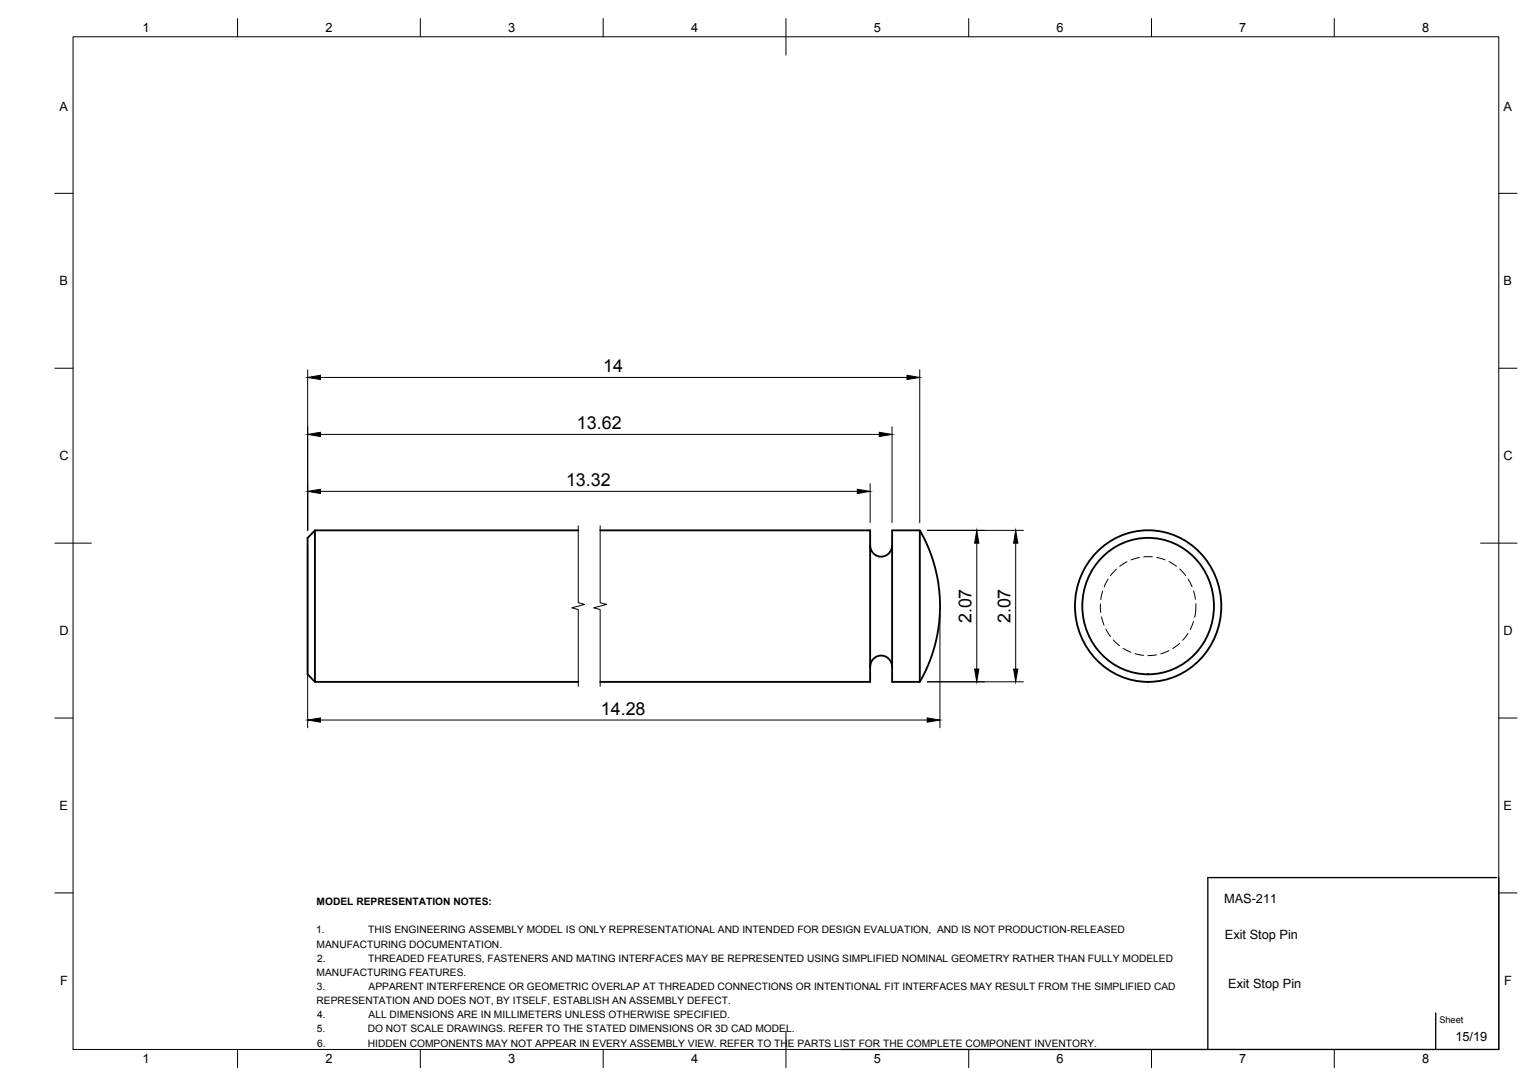
ISO-10303-21;
HEADER;
FILE_DESCRIPTION(
 (''),
 '2;1');
FILE_NAME ( 'Exit Stop Pin.step', '2026-10-05T20:07:59+06:00', ( '' ), ( '' ), 'STEP AP214', 'Unspecified', '' );
FILE_SCHEMA (('AUTOMOTIVE_DESIGN { 1 0 10303 214 3 1 1 }'));
ENDSEC;
DATA;
#10=MECHANICAL_DESIGN_GEOMETRIC_PRESENTATION_REPRESENTATION('',(#333),#196741);
#26=(
BOUNDED_CURVE()
B_SPLINE_CURVE(2,(#154684,#154685,#154686,#154687,#154688,#154689,#154690,
#154691,#154692),.UNSPECIFIED.,.F.,.F.)
B_SPLINE_CURVE_WITH_KNOTS((3,2,2,2,3),(1.42918797785348,1.62618617063892,
1.86180561965816,2.09742506867739,2.29442326146283),.UNSPECIFIED.)
CURVE()
GEOMETRIC_REPRESENTATION_ITEM()
RATIONAL_B_SPLINE_CURVE((1.,1.,1.,0.707106781186548,1.,0.707106781186548,
1.,1.,1.))
REPRESENTATION_ITEM('')
) ;
#56=(
BOUNDED_SURFACE()
B_SPLINE_SURFACE(2,2,((#154549,#154550,#154551,#154552,#154553,#154554,
#154555,#154556,#154557),(#154558,#154559,#154560,#154561,#154562,#154563,
#154564,#154565,#154566),(#154567,#154568,#154569,#154570,#154571,#154572,
#154573,#154574,#154575)),.UNSPECIFIED.,.F.,.T.,.F.)
B_SPLINE_SURFACE_WITH_KNOTS((3,3),(3,2,2,2,3),(0.,1.05013832301181),(0.,
1.5707963267949,3.1415926535898,4.71238898038469,6.28318530717959),
 .UNSPECIFIED.)
GEOMETRIC_REPRESENTATION_ITEM()
RATIONAL_B_SPLINE_SURFACE(((1.,0.707106781186548,1.,0.707106781186548,1.,
0.707106781186548,1.,0.707106781186548,1.),(0.963886720506905,0.681570836366095,
0.963886720506905,0.681570836366095,0.963886720506905,0.681570836366095,
0.963886720506905,0.681570836366095,0.963886720506905),(1.,0.707106781186548,
1.,0.707106781186548,1.,0.707106781186548,1.,0.707106781186548,1.)))
REPRESENTATION_ITEM('')
SURFACE()
) ;
#57=(
BOUNDED_SURFACE()
B_SPLINE_SURFACE(2,1,((#154580,#154581),(#154582,#154583),(#154584,#154585),
(#154586,#154587),(#154588,#154589),(#154590,#154591),(#154592,#154593),
(#154594,#154595),(#154596,#154597)),.UNSPECIFIED.,.T.,.F.,.F.)
B_SPLINE_SURFACE_WITH_KNOTS((3,2,2,2,3),(2,2),(0.,1.5707963267949,3.1415926535898,
4.71238898038469,6.28318530717959),(0.,0.0454859585810007),
 .UNSPECIFIED.)
GEOMETRIC_REPRESENTATION_ITEM()
RATIONAL_B_SPLINE_SURFACE(((1.,1.),(0.707106781186548,0.707106781186548),
(1.,1.),(0.707106781186548,0.707106781186548),(1.,1.),(0.707106781186548,
0.707106781186548),(1.,1.),(0.707106781186548,0.707106781186548),(1.,1.)))
REPRESENTATION_ITEM('')
SURFACE()
) ;
#58=(
BOUNDED_SURFACE()
B_SPLINE_SURFACE(2,2,((#154601,#154602,#154603,#154604,#154605,#154606,
#154607,#154608,#154609),(#154610,#154611,#154612,#154613,#154614,#154615,
#154616,#154617,#154618),(#154619,#154620,#154621,#154622,#154623,#154624,
#154625,#154626,#154627),(#154628,#154629,#154630,#154631,#154632,#154633,
#154634,#154635,#154636),(#154637,#154638,#154639,#154640,#154641,#154642,
#154643,#154644,#154645),(#154646,#154647,#154648,#154649,#154650,#154651,
#154652,#154653,#154654),(#154655,#154656,#154657,#154658,#154659,#154660,
#154661,#154662,#154663),(#154664,#154665,#154666,#154667,#154668,#154669,
#154670,#154671,#154672),(#154673,#154674,#154675,#154676,#154677,#154678,
#154679,#154680,#154681)),.UNSPECIFIED.,.F.,.T.,.F.)
B_SPLINE_SURFACE_WITH_KNOTS((3,2,2,2,3),(3,2,2,2,3),(1.42918797785348,1.62618617063892,
1.86180561965816,2.09742506867739,2.29442326146283),(0.,1.5707963267949,
3.1415926535898,4.71238898038469,6.28318530717959),.UNSPECIFIED.)
GEOMETRIC_REPRESENTATION_ITEM()
RATIONAL_B_SPLINE_SURFACE(((1.,0.707106781186548,1.,0.707106781186548,1.,
0.707106781186548,1.,0.707106781186548,1.),(1.,0.707106781186548,1.,0.707106781186548,
1.,0.707106781186548,1.,0.707106781186548,1.),(1.,0.707106781186548,1.,
0.707106781186548,1.,0.707106781186548,1.,0.707106781186548,1.),(0.707106781186548,
0.5,0.707106781186548,0.5,0.707106781186548,0.5,0.707106781186548,0.5,0.707106781186548),
(1.,0.707106781186548,1.,0.707106781186548,1.,0.707106781186548,1.,0.707106781186548,
1.),(0.707106781186548,0.5,0.707106781186548,0.5,0.707106781186548,0.5,
0.707106781186548,0.5,0.707106781186548),(1.,0.707106781186548,1.,0.707106781186548,
1.,0.707106781186548,1.,0.707106781186548,1.),(1.,0.707106781186548,1.,
0.707106781186548,1.,0.707106781186548,1.,0.707106781186548,1.),(1.,0.707106781186548,
1.,0.707106781186548,1.,0.707106781186548,1.,0.707106781186548,1.)))
REPRESENTATION_ITEM('')
SURFACE()
) ;
#59=(
BOUNDED_SURFACE()
B_SPLINE_SURFACE(2,1,((#154693,#154694),(#154695,#154696),(#154697,#154698),
(#154699,#154700),(#154701,#154702),(#154703,#154704),(#154705,#154706),
(#154707,#154708),(#154709,#154710)),.UNSPECIFIED.,.T.,.F.,.F.)
B_SPLINE_SURFACE_WITH_KNOTS((3,2,2,2,3),(2,2),(0.,1.5707963267949,3.1415926535898,
4.71238898038469,6.28318530717959),(0.,1.586514041419),.UNSPECIFIED.)
GEOMETRIC_REPRESENTATION_ITEM()
RATIONAL_B_SPLINE_SURFACE(((1.,1.),(0.707106781186548,0.707106781186548),
(1.,1.),(0.707106781186548,0.707106781186548),(1.,1.),(0.707106781186548,
0.707106781186548),(1.,1.),(0.707106781186548,0.707106781186548),(1.,1.)))
REPRESENTATION_ITEM('')
SURFACE()
) ;
#60=(
BOUNDED_SURFACE()
B_SPLINE_SURFACE(1,2,((#154714,#154715,#154716,#154717,#154718,#154719,
#154720,#154721,#154722),(#154723,#154724,#154725,#154726,#154727,#154728,
#154729,#154730,#154731)),.UNSPECIFIED.,.F.,.T.,.F.)
B_SPLINE_SURFACE_WITH_KNOTS((2,2),(3,2,2,2,3),(15.5153736066212,15.6567949628585),
(0.,1.5707963267949,3.1415926535898,4.71238898038469,6.28318530717959),
 .UNSPECIFIED.)
GEOMETRIC_REPRESENTATION_ITEM()
RATIONAL_B_SPLINE_SURFACE(((1.,0.707106781186548,1.,0.707106781186548,1.,
0.707106781186548,1.,0.707106781186548,1.),(1.,0.707106781186548,1.,0.707106781186548,
1.,0.707106781186548,1.,0.707106781186548,1.)))
REPRESENTATION_ITEM('')
SURFACE()
) ;
#170=ELLIPSE('',#9016,0.932157550311782,0.900000000000012) ;
#171=ELLIPSE('',#9017,1.03573061145752,1.) ;
#172=ELLIPSE('',#9019,1.03573061145752,1.) ;
#173=ELLIPSE('',#9020,1.03573061145752,1.) ;
#174=ELLIPSE('',#9021,1.03573061145752,1.) ;
#333=STYLED_ITEM('',(#196765),#352) ;
#352=MANIFOLD_SOLID_BREP('Exit Stop Pin',#8729) ;
#405=PLANE('',#9015) ;
#710=CIRCLE('',#9018,1.94783572104112) ;
#1060=FACE_OUTER_BOUND('',#1569,.T.) ;
#1061=FACE_OUTER_BOUND('',#1570,.T.) ;
#1062=FACE_OUTER_BOUND('',#1571,.T.) ;
#1063=FACE_OUTER_BOUND('',#1572,.T.) ;
#1064=FACE_OUTER_BOUND('',#1573,.T.) ;
#1065=FACE_OUTER_BOUND('',#1574,.T.) ;
#1569=EDGE_LOOP('',(#6574,#6575,#6576)) ;
#1570=EDGE_LOOP('',(#6577,#6578,#6579)) ;
#1571=EDGE_LOOP('',(#6580,#6581,#6582,#6583)) ;
#1572=EDGE_LOOP('',(#6584,#6585,#6586,#6587)) ;
#1573=EDGE_LOOP('',(#6588,#6589,#6590,#6591)) ;
#1574=EDGE_LOOP('',(#6592,#6593,#6594,#6595)) ;
#2048=LINE('',#154547,#2751) ;
#2049=LINE('',#154600,#2752) ;
#2050=LINE('',#154713,#2753) ;
#2051=LINE('',#154732,#2754) ;
#2751=VECTOR('',#10180,10.) ;
#2752=VECTOR('',#10189,10.) ;
#2753=VECTOR('',#10194,10.) ;
#2754=VECTOR('',#10195,10.) ;
#3777=VERTEX_POINT('',#154545) ;
#3778=VERTEX_POINT('',#154546) ;
#3779=VERTEX_POINT('',#154576) ;
#3780=VERTEX_POINT('',#154578) ;
#3781=VERTEX_POINT('',#154598) ;
#3782=VERTEX_POINT('',#154682) ;
#3783=VERTEX_POINT('',#154711) ;
#4795=EDGE_CURVE('',#3777,#3778,#2048,.T.) ;
#4796=EDGE_CURVE('',#3777,#3777,#170,.T.) ;
#4797=EDGE_CURVE('',#3779,#3779,#171,.T.) ;
#4798=EDGE_CURVE('',#3780,#3779,#710,.T.) ;
#4799=EDGE_CURVE('',#3781,#3781,#172,.T.) ;
#4800=EDGE_CURVE('',#3779,#3781,#2049,.T.) ;
#4801=EDGE_CURVE('',#3782,#3782,#173,.T.) ;
#4802=EDGE_CURVE('',#3781,#3782,#26,.T.) ;
#4803=EDGE_CURVE('',#3783,#3783,#174,.T.) ;
#4804=EDGE_CURVE('',#3782,#3783,#2050,.T.) ;
#4805=EDGE_CURVE('',#3783,#3777,#2051,.T.) ;
#6574=ORIENTED_EDGE('',*,*,#4795,.T.) ;
#6575=ORIENTED_EDGE('',*,*,#4795,.F.) ;
#6576=ORIENTED_EDGE('',*,*,#4796,.F.) ;
#6577=ORIENTED_EDGE('',*,*,#4797,.T.) ;
#6578=ORIENTED_EDGE('',*,*,#4798,.F.) ;
#6579=ORIENTED_EDGE('',*,*,#4798,.T.) ;
#6580=ORIENTED_EDGE('',*,*,#4799,.T.) ;
#6581=ORIENTED_EDGE('',*,*,#4800,.F.) ;
#6582=ORIENTED_EDGE('',*,*,#4797,.F.) ;
#6583=ORIENTED_EDGE('',*,*,#4800,.T.) ;
#6584=ORIENTED_EDGE('',*,*,#4801,.T.) ;
#6585=ORIENTED_EDGE('',*,*,#4802,.F.) ;
#6586=ORIENTED_EDGE('',*,*,#4799,.F.) ;
#6587=ORIENTED_EDGE('',*,*,#4802,.T.) ;
#6588=ORIENTED_EDGE('',*,*,#4803,.T.) ;
#6589=ORIENTED_EDGE('',*,*,#4804,.F.) ;
#6590=ORIENTED_EDGE('',*,*,#4801,.F.) ;
#6591=ORIENTED_EDGE('',*,*,#4804,.T.) ;
#6592=ORIENTED_EDGE('',*,*,#4796,.T.) ;
#6593=ORIENTED_EDGE('',*,*,#4805,.F.) ;
#6594=ORIENTED_EDGE('',*,*,#4803,.F.) ;
#6595=ORIENTED_EDGE('',*,*,#4805,.T.) ;
#8443=ADVANCED_FACE('',(#1060),#405,.T.) ;
#8444=ADVANCED_FACE('',(#1061),#56,.T.) ;
#8445=ADVANCED_FACE('',(#1062),#57,.F.) ;
#8446=ADVANCED_FACE('',(#1063),#58,.T.) ;
#8447=ADVANCED_FACE('',(#1064),#59,.F.) ;
#8448=ADVANCED_FACE('',(#1065),#60,.T.) ;
#8729=CLOSED_SHELL('',(#8443,#8444,#8445,#8446,#8447,#8448)) ;
#9015=AXIS2_PLACEMENT_3D('',#154544,#10178,#10179) ;
#9016=AXIS2_PLACEMENT_3D('',#154548,#10181,#10182) ;
#9017=AXIS2_PLACEMENT_3D('',#154577,#10183,#10184) ;
#9018=AXIS2_PLACEMENT_3D('',#154579,#10185,#10186) ;
#9019=AXIS2_PLACEMENT_3D('',#154599,#10187,#10188) ;
#9020=AXIS2_PLACEMENT_3D('',#154683,#10190,#10191) ;
#9021=AXIS2_PLACEMENT_3D('',#154712,#10192,#10193) ;
#10178=DIRECTION('center_axis',(0.,1.,0.)) ;
#10179=DIRECTION('ref_axis',(0.,0.,1.)) ;
#10180=DIRECTION('',(0.311934930442493,-6.02334540269699E-19,-0.950103467612784)) ;
#10181=DIRECTION('center_axis',(-5.21384921350609E-19,-1.,-8.56810894045757E-20)) ;
#10182=DIRECTION('ref_axis',(0.950103467612636,-5.22096546399847E-19,0.311934930442945)) ;
#10183=DIRECTION('center_axis',(-8.59827508034601E-16,-1.,9.95527653635857E-16)) ;
#10184=DIRECTION('ref_axis',(0.950103467612776,-5.06385247542023E-16,0.311934930442517)) ;
#10185=DIRECTION('center_axis',(-0.950103467612784,4.27867700308741E-14,
-0.311934930442494)) ;
#10186=DIRECTION('ref_axis',(-0.160144373097263,-0.858155219939135,0.487773921255021)) ;
#10187=DIRECTION('center_axis',(0.,-1.,0.)) ;
#10188=DIRECTION('ref_axis',(0.950103467612776,0.,0.311934930442517)) ;
#10189=DIRECTION('',(0.,1.,4.6863433766804E-14)) ;
#10190=DIRECTION('center_axis',(-1.92203337406689E-15,-1.,-3.15854767981034E-16)) ;
#10191=DIRECTION('ref_axis',(0.950103467612776,-1.92465670864854E-15,0.311934930442517)) ;
#10192=DIRECTION('center_axis',(0.,-1.,0.)) ;
#10193=DIRECTION('ref_axis',(0.95010346761278,0.,0.311934930442505)) ;
#10194=DIRECTION('',(0.,1.,1.34359239920357E-15)) ;
#10195=DIRECTION('',(0.220571304604875,0.707106781186631,-0.671824604777754)) ;
#154544=CARTESIAN_POINT('Origin',(-5.81917539329314,-0.00455472950331526,
120.408087607083)) ;
#154545=CARTESIAN_POINT('',(-5.95954611199226,-0.00455472950331526,120.835634167509)) ;
#154546=CARTESIAN_POINT('',(-5.67880467459401,-0.00455472950331526,119.980541046657)) ;
#154547=CARTESIAN_POINT('',(-5.95954611199226,-0.00455472950331526,120.835634167509)) ;
#154548=CARTESIAN_POINT('Origin',(-5.67880467459401,-0.00455472950331526,
119.980541046657)) ;
#154549=CARTESIAN_POINT('Ctrl Pts',(-5.67880467459401,-14.2808450589491,
119.980541046657)) ;
#154550=CARTESIAN_POINT('Ctrl Pts',(-5.67880467459401,-14.2808450589491,
119.980541046657)) ;
#154551=CARTESIAN_POINT('Ctrl Pts',(-5.67880467459401,-14.2808450589491,
119.980541046657)) ;
#154552=CARTESIAN_POINT('Ctrl Pts',(-5.67880467459401,-14.2808450589491,
119.980541046657)) ;
#154553=CARTESIAN_POINT('Ctrl Pts',(-5.67880467459401,-14.2808450589491,
119.980541046657)) ;
#154554=CARTESIAN_POINT('Ctrl Pts',(-5.67880467459401,-14.2808450589491,
119.980541046657)) ;
#154555=CARTESIAN_POINT('Ctrl Pts',(-5.67880467459401,-14.2808450589491,
119.980541046657)) ;
#154556=CARTESIAN_POINT('Ctrl Pts',(-5.67880467459401,-14.2808450589491,
119.980541046657)) ;
#154557=CARTESIAN_POINT('Ctrl Pts',(-5.67880467459401,-14.2808450589491,
119.980541046657)) ;
#154558=CARTESIAN_POINT('Ctrl Pts',(-5.84667812622779,-14.2808450589491,
120.491856494052)) ;
#154559=CARTESIAN_POINT('Ctrl Pts',(-6.37626318720601,-14.2808450589491,
120.317984821344)) ;
#154560=CARTESIAN_POINT('Ctrl Pts',(-6.20838973557223,-14.2808450589491,
119.806669373949)) ;
#154561=CARTESIAN_POINT('Ctrl Pts',(-6.04051628393846,-14.2808450589491,
119.295353926554)) ;
#154562=CARTESIAN_POINT('Ctrl Pts',(-5.51093122296023,-14.2808450589491,
119.469225599262)) ;
#154563=CARTESIAN_POINT('Ctrl Pts',(-4.981346161982,-14.2808450589491,119.64309727197)) ;
#154564=CARTESIAN_POINT('Ctrl Pts',(-5.14921961361578,-14.2808450589491,
120.154412719365)) ;
#154565=CARTESIAN_POINT('Ctrl Pts',(-5.31709306524956,-14.2808450589491,
120.66572816676)) ;
#154566=CARTESIAN_POINT('Ctrl Pts',(-5.84667812622779,-14.2808450589491,
120.491856494052)) ;
#154567=CARTESIAN_POINT('Ctrl Pts',(-5.99073960503651,-14.0045547295033,
120.93064451427)) ;
#154568=CARTESIAN_POINT('Ctrl Pts',(-6.97479085049501,-14.0045547295033,
120.607563958028)) ;
#154569=CARTESIAN_POINT('Ctrl Pts',(-6.6628559200525,-14.0045547295033,
119.657460490415)) ;
#154570=CARTESIAN_POINT('Ctrl Pts',(-6.35092098961,-14.0045547295033,118.707357022802)) ;
#154571=CARTESIAN_POINT('Ctrl Pts',(-5.36686974415151,-14.0045547295033,
119.030437579044)) ;
#154572=CARTESIAN_POINT('Ctrl Pts',(-4.38281849869301,-14.0045547295033,
119.353518135287)) ;
#154573=CARTESIAN_POINT('Ctrl Pts',(-4.69475342913551,-14.0045547295033,
120.303621602899)) ;
#154574=CARTESIAN_POINT('Ctrl Pts',(-5.00668835957801,-14.0045547295033,
121.253725070512)) ;
#154575=CARTESIAN_POINT('Ctrl Pts',(-5.99073960503651,-14.0045547295033,
120.93064451427)) ;
#154576=CARTESIAN_POINT('',(-5.99073960503651,-14.0045547295033,120.93064451427)) ;
#154577=CARTESIAN_POINT('Origin',(-5.67880467459401,-14.0045547295033,119.980541046657)) ;
#154578=CARTESIAN_POINT('',(-5.67880467459401,-14.2808450589491,119.980541046657)) ;
#154579=CARTESIAN_POINT('Origin',(-5.67880467459393,-12.333009337908,119.980541046657)) ;
#154580=CARTESIAN_POINT('Ctrl Pts',(-5.99073960503651,-14.0045547295033,
120.93064451427)) ;
#154581=CARTESIAN_POINT('Ctrl Pts',(-5.99073960503651,-13.5496951436933,
120.93064451427)) ;
#154582=CARTESIAN_POINT('Ctrl Pts',(-6.97479085049501,-14.0045547295033,
120.607563958028)) ;
#154583=CARTESIAN_POINT('Ctrl Pts',(-6.97479085049501,-13.5496951436933,
120.607563958028)) ;
#154584=CARTESIAN_POINT('Ctrl Pts',(-6.6628559200525,-14.0045547295033,
119.657460490415)) ;
#154585=CARTESIAN_POINT('Ctrl Pts',(-6.6628559200525,-13.5496951436933,
119.657460490415)) ;
#154586=CARTESIAN_POINT('Ctrl Pts',(-6.35092098961,-14.0045547295033,118.707357022802)) ;
#154587=CARTESIAN_POINT('Ctrl Pts',(-6.35092098961,-13.5496951436933,118.707357022802)) ;
#154588=CARTESIAN_POINT('Ctrl Pts',(-5.3668697441515,-14.0045547295033,
119.030437579044)) ;
#154589=CARTESIAN_POINT('Ctrl Pts',(-5.3668697441515,-13.5496951436933,
119.030437579044)) ;
#154590=CARTESIAN_POINT('Ctrl Pts',(-4.38281849869301,-14.0045547295033,
119.353518135287)) ;
#154591=CARTESIAN_POINT('Ctrl Pts',(-4.38281849869301,-13.5496951436933,
119.353518135287)) ;
#154592=CARTESIAN_POINT('Ctrl Pts',(-4.69475342913551,-14.0045547295033,
120.303621602899)) ;
#154593=CARTESIAN_POINT('Ctrl Pts',(-4.69475342913551,-13.5496951436933,
120.303621602899)) ;
#154594=CARTESIAN_POINT('Ctrl Pts',(-5.00668835957802,-14.0045547295033,
121.253725070512)) ;
#154595=CARTESIAN_POINT('Ctrl Pts',(-5.00668835957802,-13.5496951436933,
121.253725070512)) ;
#154596=CARTESIAN_POINT('Ctrl Pts',(-5.99073960503651,-14.0045547295033,
120.93064451427)) ;
#154597=CARTESIAN_POINT('Ctrl Pts',(-5.99073960503651,-13.5496951436933,
120.93064451427)) ;
#154598=CARTESIAN_POINT('',(-5.99073960503651,-13.6255050746616,120.93064451427)) ;
#154599=CARTESIAN_POINT('Origin',(-5.67880467459401,-13.6255050746616,119.980541046657)) ;
#154600=CARTESIAN_POINT('',(-5.99073960503651,-14.0045547295033,120.93064451427)) ;
#154601=CARTESIAN_POINT('Ctrl Pts',(-5.99073960503651,-13.6255050746616,
120.93064451427)) ;
#154602=CARTESIAN_POINT('Ctrl Pts',(-6.97479085049501,-13.6255050746616,
120.607563958028)) ;
#154603=CARTESIAN_POINT('Ctrl Pts',(-6.6628559200525,-13.6255050746616,
119.657460490415)) ;
#154604=CARTESIAN_POINT('Ctrl Pts',(-6.35092098961,-13.6255050746616,118.707357022802)) ;
#154605=CARTESIAN_POINT('Ctrl Pts',(-5.3668697441515,-13.6255050746616,
119.030437579044)) ;
#154606=CARTESIAN_POINT('Ctrl Pts',(-4.38281849869301,-13.6255050746616,
119.353518135287)) ;
#154607=CARTESIAN_POINT('Ctrl Pts',(-4.69475342913551,-13.6255050746616,
120.303621602899)) ;
#154608=CARTESIAN_POINT('Ctrl Pts',(-5.00668835957802,-13.6255050746616,
121.253725070512)) ;
#154609=CARTESIAN_POINT('Ctrl Pts',(-5.99073960503651,-13.6255050746616,
120.93064451427)) ;
#154610=CARTESIAN_POINT('Ctrl Pts',(-5.9600142962546,-13.6255050746616,
120.837060181231)) ;
#154611=CARTESIAN_POINT('Ctrl Pts',(-6.84713738323131,-13.6255050746616,
120.54580276784)) ;
#154612=CARTESIAN_POINT('Ctrl Pts',(-6.56592776157072,-13.6255050746616,
119.689283633267)) ;
#154613=CARTESIAN_POINT('Ctrl Pts',(-6.28471813991013,-13.6255050746616,
118.832764498694)) ;
#154614=CARTESIAN_POINT('Ctrl Pts',(-5.39759505293342,-13.6255050746616,
119.124021912084)) ;
#154615=CARTESIAN_POINT('Ctrl Pts',(-4.51047196595671,-13.6255050746616,
119.415279325474)) ;
#154616=CARTESIAN_POINT('Ctrl Pts',(-4.7916815876173,-13.6255050746616,
120.271798460047)) ;
#154617=CARTESIAN_POINT('Ctrl Pts',(-5.07289120927789,-13.6255050746616,
121.128317594621)) ;
#154618=CARTESIAN_POINT('Ctrl Pts',(-5.9600142962546,-13.6255050746616,
120.837060181231)) ;
#154619=CARTESIAN_POINT('Ctrl Pts',(-5.92928898747268,-13.6255050746616,
120.743475848191)) ;
#154620=CARTESIAN_POINT('Ctrl Pts',(-6.71948391596759,-13.6255050746616,
120.484041577653)) ;
#154621=CARTESIAN_POINT('Ctrl Pts',(-6.46899960308891,-13.6255050746616,
119.721106776119)) ;
#154622=CARTESIAN_POINT('Ctrl Pts',(-6.21851529021024,-13.6255050746616,
118.958171974585)) ;
#154623=CARTESIAN_POINT('Ctrl Pts',(-5.42832036171533,-13.6255050746616,
119.217606245123)) ;
#154624=CARTESIAN_POINT('Ctrl Pts',(-4.63812543322043,-13.6255050746616,
119.477040515662)) ;
#154625=CARTESIAN_POINT('Ctrl Pts',(-4.8886097460991,-13.6255050746616,
120.239975317196)) ;
#154626=CARTESIAN_POINT('Ctrl Pts',(-5.13909405897778,-13.6255050746616,
121.002910118729)) ;
#154627=CARTESIAN_POINT('Ctrl Pts',(-5.92928898747268,-13.6255050746616,
120.743475848191)) ;
#154628=CARTESIAN_POINT('Ctrl Pts',(-5.88249874790631,-13.6255050746616,
120.600960328049)) ;
#154629=CARTESIAN_POINT('Ctrl Pts',(-6.52508598958243,-13.6255050746616,
120.389988140947)) ;
#154630=CARTESIAN_POINT('Ctrl Pts',(-6.32139191627013,-13.6255050746616,
119.769568859555)) ;
#154631=CARTESIAN_POINT('Ctrl Pts',(-6.11769784295783,-13.6255050746616,
119.149149578163)) ;
#154632=CARTESIAN_POINT('Ctrl Pts',(-5.47511060128171,-13.6255050746616,
119.360121765265)) ;
#154633=CARTESIAN_POINT('Ctrl Pts',(-4.83252335960559,-13.6255050746616,
119.571093952367)) ;
#154634=CARTESIAN_POINT('Ctrl Pts',(-5.03621743291789,-13.6255050746616,
120.191513233759)) ;
#154635=CARTESIAN_POINT('Ctrl Pts',(-5.23991150623019,-13.6255050746616,
120.811932515151)) ;
#154636=CARTESIAN_POINT('Ctrl Pts',(-5.88249874790631,-13.6255050746616,
120.600960328049)) ;
#154637=CARTESIAN_POINT('Ctrl Pts',(-5.88249874790631,-13.4755050746616,
120.600960328049)) ;
#154638=CARTESIAN_POINT('Ctrl Pts',(-6.52508598958244,-13.4755050746616,
120.389988140947)) ;
#154639=CARTESIAN_POINT('Ctrl Pts',(-6.32139191627014,-13.4755050746616,
119.769568859555)) ;
#154640=CARTESIAN_POINT('Ctrl Pts',(-6.11769784295784,-13.4755050746616,
119.149149578163)) ;
#154641=CARTESIAN_POINT('Ctrl Pts',(-5.47511060128171,-13.4755050746616,
119.360121765265)) ;
#154642=CARTESIAN_POINT('Ctrl Pts',(-4.83252335960557,-13.4755050746616,
119.571093952367)) ;
#154643=CARTESIAN_POINT('Ctrl Pts',(-5.03621743291787,-13.4755050746616,
120.191513233759)) ;
#154644=CARTESIAN_POINT('Ctrl Pts',(-5.23991150623018,-13.4755050746616,
120.811932515151)) ;
#154645=CARTESIAN_POINT('Ctrl Pts',(-5.88249874790631,-13.4755050746616,
120.600960328049)) ;
#154646=CARTESIAN_POINT('Ctrl Pts',(-5.88249874790631,-13.3255050746616,
120.600960328049)) ;
#154647=CARTESIAN_POINT('Ctrl Pts',(-6.52508598958243,-13.3255050746616,
120.389988140947)) ;
#154648=CARTESIAN_POINT('Ctrl Pts',(-6.32139191627013,-13.3255050746616,
119.769568859555)) ;
#154649=CARTESIAN_POINT('Ctrl Pts',(-6.11769784295783,-13.3255050746616,
119.149149578163)) ;
#154650=CARTESIAN_POINT('Ctrl Pts',(-5.47511060128171,-13.3255050746616,
119.360121765265)) ;
#154651=CARTESIAN_POINT('Ctrl Pts',(-4.83252335960559,-13.3255050746616,
119.571093952367)) ;
#154652=CARTESIAN_POINT('Ctrl Pts',(-5.03621743291789,-13.3255050746616,
120.191513233759)) ;
#154653=CARTESIAN_POINT('Ctrl Pts',(-5.23991150623019,-13.3255050746616,
120.811932515151)) ;
#154654=CARTESIAN_POINT('Ctrl Pts',(-5.88249874790631,-13.3255050746616,
120.600960328049)) ;
#154655=CARTESIAN_POINT('Ctrl Pts',(-5.92928898747268,-13.3255050746616,
120.743475848191)) ;
#154656=CARTESIAN_POINT('Ctrl Pts',(-6.71948391596759,-13.3255050746616,
120.484041577653)) ;
#154657=CARTESIAN_POINT('Ctrl Pts',(-6.46899960308891,-13.3255050746616,
119.721106776119)) ;
#154658=CARTESIAN_POINT('Ctrl Pts',(-6.21851529021024,-13.3255050746616,
118.958171974585)) ;
#154659=CARTESIAN_POINT('Ctrl Pts',(-5.42832036171533,-13.3255050746616,
119.217606245123)) ;
#154660=CARTESIAN_POINT('Ctrl Pts',(-4.63812543322043,-13.3255050746616,
119.477040515662)) ;
#154661=CARTESIAN_POINT('Ctrl Pts',(-4.8886097460991,-13.3255050746616,
120.239975317196)) ;
#154662=CARTESIAN_POINT('Ctrl Pts',(-5.13909405897778,-13.3255050746616,
121.002910118729)) ;
#154663=CARTESIAN_POINT('Ctrl Pts',(-5.92928898747268,-13.3255050746616,
120.743475848191)) ;
#154664=CARTESIAN_POINT('Ctrl Pts',(-5.9600142962546,-13.3255050746616,
120.837060181231)) ;
#154665=CARTESIAN_POINT('Ctrl Pts',(-6.84713738323131,-13.3255050746616,
120.54580276784)) ;
#154666=CARTESIAN_POINT('Ctrl Pts',(-6.56592776157072,-13.3255050746616,
119.689283633267)) ;
#154667=CARTESIAN_POINT('Ctrl Pts',(-6.28471813991013,-13.3255050746616,
118.832764498694)) ;
#154668=CARTESIAN_POINT('Ctrl Pts',(-5.39759505293342,-13.3255050746616,
119.124021912084)) ;
#154669=CARTESIAN_POINT('Ctrl Pts',(-4.51047196595671,-13.3255050746616,
119.415279325474)) ;
#154670=CARTESIAN_POINT('Ctrl Pts',(-4.7916815876173,-13.3255050746616,
120.271798460047)) ;
#154671=CARTESIAN_POINT('Ctrl Pts',(-5.07289120927789,-13.3255050746616,
121.128317594621)) ;
#154672=CARTESIAN_POINT('Ctrl Pts',(-5.9600142962546,-13.3255050746616,
120.837060181231)) ;
#154673=CARTESIAN_POINT('Ctrl Pts',(-5.99073960503651,-13.3255050746616,
120.93064451427)) ;
#154674=CARTESIAN_POINT('Ctrl Pts',(-6.97479085049501,-13.3255050746616,
120.607563958028)) ;
#154675=CARTESIAN_POINT('Ctrl Pts',(-6.6628559200525,-13.3255050746616,
119.657460490415)) ;
#154676=CARTESIAN_POINT('Ctrl Pts',(-6.35092098961,-13.3255050746616,118.707357022802)) ;
#154677=CARTESIAN_POINT('Ctrl Pts',(-5.3668697441515,-13.3255050746616,
119.030437579044)) ;
#154678=CARTESIAN_POINT('Ctrl Pts',(-4.38281849869301,-13.3255050746616,
119.353518135287)) ;
#154679=CARTESIAN_POINT('Ctrl Pts',(-4.69475342913551,-13.3255050746616,
120.303621602899)) ;
#154680=CARTESIAN_POINT('Ctrl Pts',(-5.00668835957802,-13.3255050746616,
121.253725070512)) ;
#154681=CARTESIAN_POINT('Ctrl Pts',(-5.99073960503651,-13.3255050746616,
120.93064451427)) ;
#154682=CARTESIAN_POINT('',(-5.99073960503651,-13.3255050746616,120.93064451427)) ;
#154683=CARTESIAN_POINT('Origin',(-5.67880467459401,-13.3255050746616,119.980541046657)) ;
#154684=CARTESIAN_POINT('Ctrl Pts',(-5.99073960503651,-13.6255050746616,
120.93064451427)) ;
#154685=CARTESIAN_POINT('Ctrl Pts',(-5.9600142962546,-13.6255050746616,
120.837060181231)) ;
#154686=CARTESIAN_POINT('Ctrl Pts',(-5.92928898747268,-13.6255050746616,
120.743475848191)) ;
#154687=CARTESIAN_POINT('Ctrl Pts',(-5.88249874790631,-13.6255050746616,
120.600960328049)) ;
#154688=CARTESIAN_POINT('Ctrl Pts',(-5.88249874790631,-13.4755050746616,
120.600960328049)) ;
#154689=CARTESIAN_POINT('Ctrl Pts',(-5.88249874790631,-13.3255050746616,
120.600960328049)) ;
#154690=CARTESIAN_POINT('Ctrl Pts',(-5.92928898747268,-13.3255050746616,
120.743475848191)) ;
#154691=CARTESIAN_POINT('Ctrl Pts',(-5.9600142962546,-13.3255050746616,
120.837060181231)) ;
#154692=CARTESIAN_POINT('Ctrl Pts',(-5.99073960503651,-13.3255050746616,
120.93064451427)) ;
#154693=CARTESIAN_POINT('Ctrl Pts',(-5.99073960503651,-13.3255050746616,
120.93064451427)) ;
#154694=CARTESIAN_POINT('Ctrl Pts',(-5.99073960503651,2.53963533952835,
120.93064451427)) ;
#154695=CARTESIAN_POINT('Ctrl Pts',(-6.97479085049501,-13.3255050746616,
120.607563958028)) ;
#154696=CARTESIAN_POINT('Ctrl Pts',(-6.97479085049501,2.53963533952835,
120.607563958028)) ;
#154697=CARTESIAN_POINT('Ctrl Pts',(-6.6628559200525,-13.3255050746616,
119.657460490415)) ;
#154698=CARTESIAN_POINT('Ctrl Pts',(-6.6628559200525,2.53963533952835,119.657460490415)) ;
#154699=CARTESIAN_POINT('Ctrl Pts',(-6.35092098961,-13.3255050746616,118.707357022802)) ;
#154700=CARTESIAN_POINT('Ctrl Pts',(-6.35092098961,2.53963533952835,118.707357022802)) ;
#154701=CARTESIAN_POINT('Ctrl Pts',(-5.3668697441515,-13.3255050746616,
119.030437579044)) ;
#154702=CARTESIAN_POINT('Ctrl Pts',(-5.3668697441515,2.53963533952835,119.030437579044)) ;
#154703=CARTESIAN_POINT('Ctrl Pts',(-4.38281849869301,-13.3255050746616,
119.353518135287)) ;
#154704=CARTESIAN_POINT('Ctrl Pts',(-4.38281849869301,2.53963533952835,
119.353518135287)) ;
#154705=CARTESIAN_POINT('Ctrl Pts',(-4.69475342913551,-13.3255050746616,
120.303621602899)) ;
#154706=CARTESIAN_POINT('Ctrl Pts',(-4.69475342913551,2.53963533952835,
120.303621602899)) ;
#154707=CARTESIAN_POINT('Ctrl Pts',(-5.00668835957802,-13.3255050746616,
121.253725070512)) ;
#154708=CARTESIAN_POINT('Ctrl Pts',(-5.00668835957802,2.53963533952835,
121.253725070512)) ;
#154709=CARTESIAN_POINT('Ctrl Pts',(-5.99073960503651,-13.3255050746616,
120.93064451427)) ;
#154710=CARTESIAN_POINT('Ctrl Pts',(-5.99073960503651,2.53963533952835,
120.93064451427)) ;
#154711=CARTESIAN_POINT('',(-5.99073960503651,-0.104554729503315,120.93064451427)) ;
#154712=CARTESIAN_POINT('Origin',(-5.67880467459401,-0.104554729503315,
119.980541046657)) ;
#154713=CARTESIAN_POINT('',(-5.99073960503651,-13.3255050746616,120.93064451427)) ;
#154714=CARTESIAN_POINT('Ctrl Pts',(-5.99073960503651,-0.104554729503315,
120.93064451427)) ;
#154715=CARTESIAN_POINT('Ctrl Pts',(-6.97479085049501,-0.104554729503315,
120.607563958028)) ;
#154716=CARTESIAN_POINT('Ctrl Pts',(-6.6628559200525,-0.104554729503315,
119.657460490415)) ;
#154717=CARTESIAN_POINT('Ctrl Pts',(-6.35092098961,-0.104554729503315,118.707357022802)) ;
#154718=CARTESIAN_POINT('Ctrl Pts',(-5.3668697441515,-0.104554729503315,
119.030437579044)) ;
#154719=CARTESIAN_POINT('Ctrl Pts',(-4.38281849869301,-0.104554729503315,
119.353518135287)) ;
#154720=CARTESIAN_POINT('Ctrl Pts',(-4.69475342913551,-0.104554729503315,
120.303621602899)) ;
#154721=CARTESIAN_POINT('Ctrl Pts',(-5.00668835957802,-0.104554729503315,
121.253725070512)) ;
#154722=CARTESIAN_POINT('Ctrl Pts',(-5.99073960503651,-0.104554729503315,
120.93064451427)) ;
#154723=CARTESIAN_POINT('Ctrl Pts',(-5.95954611199226,-0.00455472950331526,
120.835634167509)) ;
#154724=CARTESIAN_POINT('Ctrl Pts',(-6.8451922329049,-0.00455472950331526,
120.544861666891)) ;
#154725=CARTESIAN_POINT('Ctrl Pts',(-6.56445079550665,-0.00455472950331526,
119.689768546039)) ;
#154726=CARTESIAN_POINT('Ctrl Pts',(-6.28370935810839,-0.00455472950331526,
118.834675425188)) ;
#154727=CARTESIAN_POINT('Ctrl Pts',(-5.39806323719575,-0.00455472950331526,
119.125447925806)) ;
#154728=CARTESIAN_POINT('Ctrl Pts',(-4.51241711628311,-0.00455472950331526,
119.416220426424)) ;
#154729=CARTESIAN_POINT('Ctrl Pts',(-4.79315855368137,-0.00455472950331526,
120.271313547275)) ;
#154730=CARTESIAN_POINT('Ctrl Pts',(-5.07389999107962,-0.00455472950331526,
121.126406668127)) ;
#154731=CARTESIAN_POINT('Ctrl Pts',(-5.95954611199226,-0.00455472950331526,
120.835634167509)) ;
#154732=CARTESIAN_POINT('',(-5.99073960503651,-0.104554729503315,120.93064451427)) ;
#196737=UNCERTAINTY_MEASURE_WITH_UNIT(LENGTH_MEASURE(0.01),#196742,
'DISTANCE_ACCURACY_VALUE',
'Maximum model space distance between geometric entities at asserted c
onnectivities') ;
#196738=UNCERTAINTY_MEASURE_WITH_UNIT(LENGTH_MEASURE(0.01),#196742,
'DISTANCE_ACCURACY_VALUE',
'Maximum model space distance between geometric entities at asserted c
onnectivities') ;
#196740=(
GEOMETRIC_REPRESENTATION_CONTEXT(3)
GLOBAL_UNCERTAINTY_ASSIGNED_CONTEXT((#196737))
GLOBAL_UNIT_ASSIGNED_CONTEXT((#196742,#196744,#196745))
REPRESENTATION_CONTEXT('','3D')
) ;
#196741=(
GEOMETRIC_REPRESENTATION_CONTEXT(3)
GLOBAL_UNCERTAINTY_ASSIGNED_CONTEXT((#196738))
GLOBAL_UNIT_ASSIGNED_CONTEXT((#196742,#196744,#196745))
REPRESENTATION_CONTEXT('','3D')
) ;
#196742=(
LENGTH_UNIT()
NAMED_UNIT(*)
SI_UNIT(.MILLI.,.METRE.)
) ;
#196744=(
NAMED_UNIT(*)
PLANE_ANGLE_UNIT()
SI_UNIT($,.RADIAN.)
) ;
#196745=(
NAMED_UNIT(*)
SI_UNIT($,.STERADIAN.)
SOLID_ANGLE_UNIT()
) ;
#196753=PRODUCT_DEFINITION_CONTEXT('part definition',#196761,'design') ;
#196761=APPLICATION_CONTEXT(
'Core Data for Automotive Mechanical Design Process') ;
#196762=PRODUCT_CONTEXT('part definition',#196761,'mechanical') ;
#196765=PRESENTATION_STYLE_ASSIGNMENT((#196767)) ;
#196767=SURFACE_STYLE_USAGE(.BOTH.,#196769) ;
#196769=SURFACE_SIDE_STYLE('',(#196771)) ;
#196771=SURFACE_STYLE_FILL_AREA(#196773) ;
#196773=FILL_AREA_STYLE('Steel - Satin',(#196775)) ;
#196775=FILL_AREA_STYLE_COLOUR('Steel - Satin',#196777) ;
#196777=COLOUR_RGB('Steel - Satin', 0.09019608, 0.27058824, 0.51372549) ;
#197115=CARTESIAN_POINT ( '', ( 0.0, 0.0, 0.0 ) ) ;
#197116=DIRECTION ( '', ( 0.0, 0.0, 1.0 ) ) ;
#197117=DIRECTION ( '', ( 1.0, 0.0, 0.0 ) ) ;
#197118=AXIS2_PLACEMENT_3D ( '', #197115, #197116, #197117 ) ;
#197119=ADVANCED_BREP_SHAPE_REPRESENTATION ( 'Exit Stop Pin', ( #352, #197118, #197129, #197420 ), #196740 ) ;
#197120=PRODUCT( 'Exit Stop Pin', 'Exit Stop Pin', '', ( #196762 ) ) ;
#197121=PRODUCT_DEFINITION_FORMATION ( '', '', #197120 ) ;
#197122=PRODUCT_DEFINITION( 'Exit Stop Pin', 'Exit Stop Pin', #197121, #196753 ) ;
#197123=PRODUCT_DEFINITION_SHAPE ( '', '', #197122 ) ;
#197124=SHAPE_DEFINITION_REPRESENTATION ( #197123, #197119 ) ;
#197126=CARTESIAN_POINT ( '', ( 0.0, 0.0, 0.0 ) ) ;
#197127=DIRECTION ( '', ( 0.0, 0.0, 1.0 ) ) ;
#197128=DIRECTION ( '', ( 1.0, 0.0, 0.0 ) ) ;
#197129=AXIS2_PLACEMENT_3D ( '', #197126, #197127, #197128 ) ;
#197417=CARTESIAN_POINT ( '', ( 0.0, 0.0, 0.0 ) ) ;
#197418=DIRECTION ( '', ( 0.0, 0.0, 1.0 ) ) ;
#197419=DIRECTION ( '', ( 1.0, 0.0, 0.0 ) ) ;
#197420=AXIS2_PLACEMENT_3D ( '', #197417, #197418, #197419 ) ;
ENDSEC;
END-ISO-10303-21;
